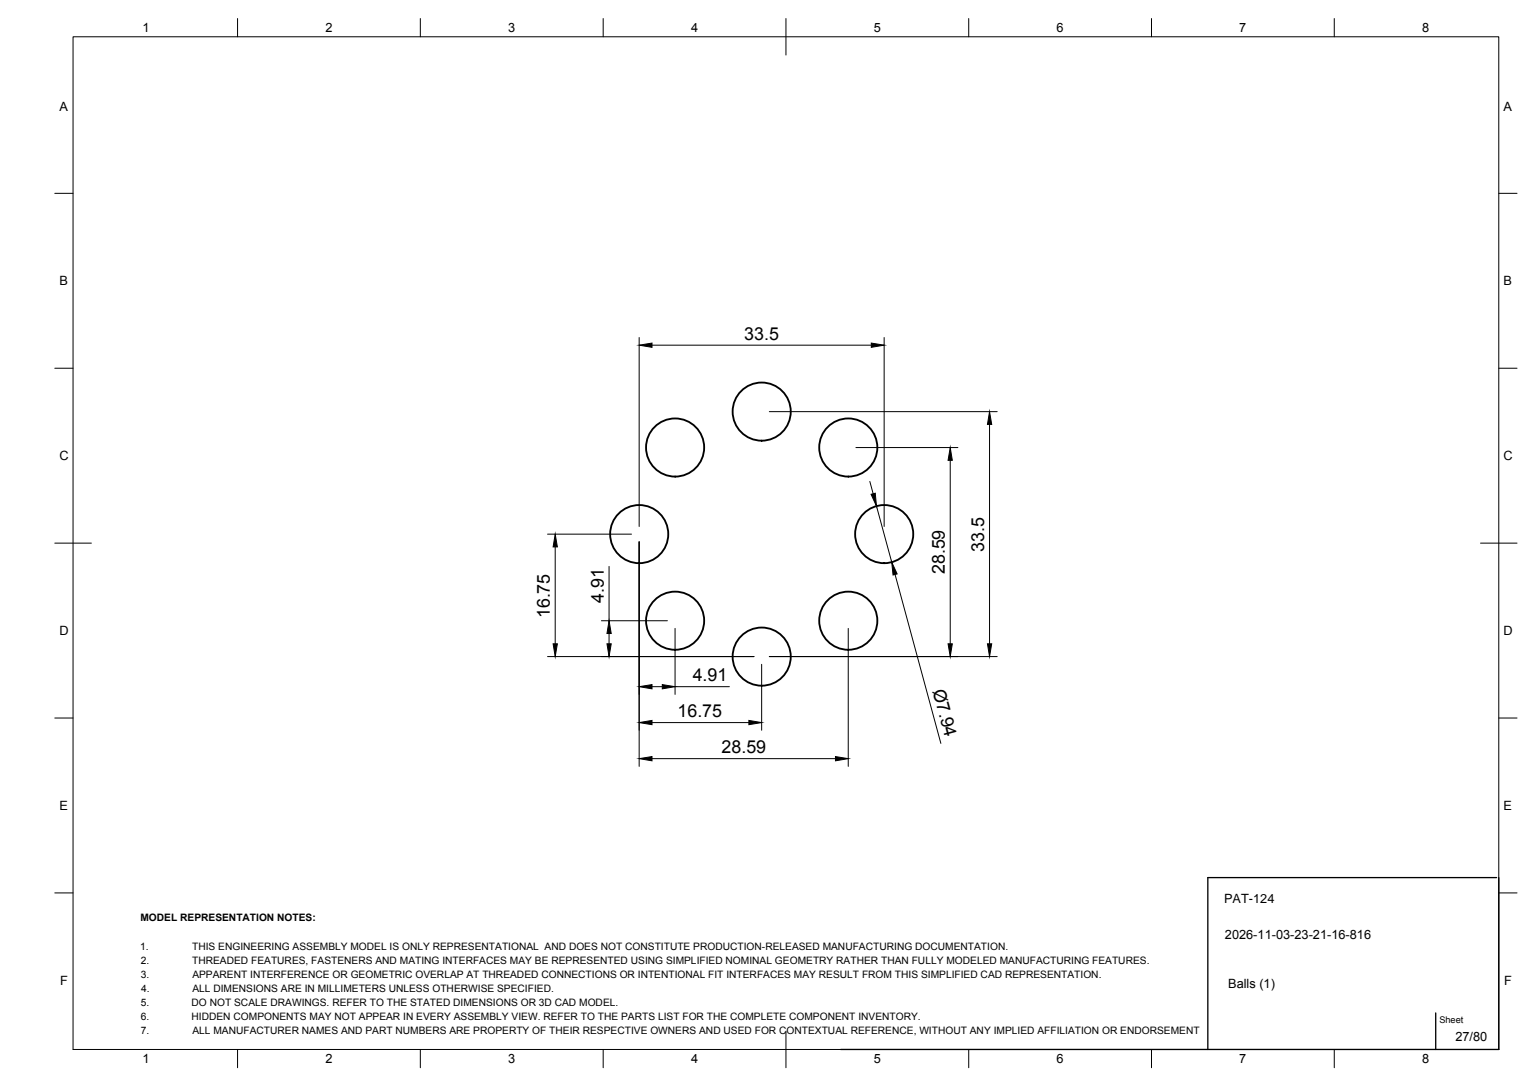
ISO-10303-21;
HEADER;
/* Generated by software containing ST-Developer
 * from STEP Tools, Inc. (www.steptools.com) 
 */

FILE_DESCRIPTION(
/* description */ ('XY cross-slide table'),
/* implementation_level */ '2;1');

FILE_NAME(
/* name */ 'Balls (1).step',
/* time_stamp */ '2026-10-28T03:22:46-07:00',
/* author */ (''),
/* organization */ (''),
/* preprocessor_version */ 'ST-DEVELOPER v20.2',
/* originating_system */ 'Autodesk Translation Framework v15.17.0.0',
/* authorisation */ '');

FILE_SCHEMA (('AUTOMOTIVE_DESIGN { 1 0 10303 214 3 1 1 }'));
ENDSEC;

DATA;
#10=MECHANICAL_DESIGN_GEOMETRIC_PRESENTATION_REPRESENTATION('',(#1695,#1696,#1697,#1698,#1699,#1700,#1701,#1702),#62984);
#1395=SPHERICAL_SURFACE('',#24455,0.3969);
#1396=SPHERICAL_SURFACE('',#24457,0.3969);
#1397=SPHERICAL_SURFACE('',#24459,0.3969);
#1398=SPHERICAL_SURFACE('',#24461,0.3969);
#1399=SPHERICAL_SURFACE('',#24463,0.3969);
#1400=SPHERICAL_SURFACE('',#24465,0.3969);
#1401=SPHERICAL_SURFACE('',#24467,0.3969);
#1402=SPHERICAL_SURFACE('',#24469,0.3969);
#1522=SHAPE_REPRESENTATION_RELATIONSHIP('SRR','None',#63372,#1605);
#1605=ADVANCED_BREP_SHAPE_REPRESENTATION('',(#1808,#1809,#1810,#1811,#1812,
#1813,#1814,#1815),#62909);
#1695=STYLED_ITEM('',(#63912),#1808);
#1696=STYLED_ITEM('',(#63912),#1809);
#1697=STYLED_ITEM('',(#63912),#1810);
#1698=STYLED_ITEM('',(#63912),#1811);
#1699=STYLED_ITEM('',(#63912),#1812);
#1700=STYLED_ITEM('',(#63912),#1813);
#1701=STYLED_ITEM('',(#63912),#1814);
#1702=STYLED_ITEM('',(#63912),#1815);
#1808=MANIFOLD_SOLID_BREP('Body1',#22989);
#1809=MANIFOLD_SOLID_BREP('Body2',#22990);
#1810=MANIFOLD_SOLID_BREP('Body3',#22991);
#1811=MANIFOLD_SOLID_BREP('Body4',#22992);
#1812=MANIFOLD_SOLID_BREP('Body5',#22993);
#1813=MANIFOLD_SOLID_BREP('Body6',#22994);
#1814=MANIFOLD_SOLID_BREP('Body7',#22995);
#1815=MANIFOLD_SOLID_BREP('Body8',#22996);
#3080=FACE_OUTER_BOUND('',#4503,.T.);
#3081=FACE_OUTER_BOUND('',#4504,.T.);
#3082=FACE_OUTER_BOUND('',#4505,.T.);
#3083=FACE_OUTER_BOUND('',#4506,.T.);
#3084=FACE_OUTER_BOUND('',#4507,.T.);
#3085=FACE_OUTER_BOUND('',#4508,.T.);
#3086=FACE_OUTER_BOUND('',#4509,.T.);
#3087=FACE_OUTER_BOUND('',#4510,.T.);
#4503=EDGE_LOOP('',(#15816,#15817));
#4504=EDGE_LOOP('',(#15818,#15819));
#4505=EDGE_LOOP('',(#15820,#15821));
#4506=EDGE_LOOP('',(#15822,#15823));
#4507=EDGE_LOOP('',(#15824,#15825));
#4508=EDGE_LOOP('',(#15826,#15827));
#4509=EDGE_LOOP('',(#15828,#15829));
#4510=EDGE_LOOP('',(#15830,#15831));
#9095=CIRCLE('',#24456,0.3969);
#9096=CIRCLE('',#24458,0.3969);
#9097=CIRCLE('',#24460,0.3969);
#9098=CIRCLE('',#24462,0.3969);
#9099=CIRCLE('',#24464,0.3969);
#9100=CIRCLE('',#24466,0.3969);
#9101=CIRCLE('',#24468,0.3969);
#9102=CIRCLE('',#24470,0.3969);
#10081=VERTEX_POINT('',#34169);
#10082=VERTEX_POINT('',#34170);
#10083=VERTEX_POINT('',#34173);
#10084=VERTEX_POINT('',#34174);
#10085=VERTEX_POINT('',#34177);
#10086=VERTEX_POINT('',#34178);
#10087=VERTEX_POINT('',#34181);
#10088=VERTEX_POINT('',#34182);
#10089=VERTEX_POINT('',#34185);
#10090=VERTEX_POINT('',#34186);
#10091=VERTEX_POINT('',#34189);
#10092=VERTEX_POINT('',#34190);
#10093=VERTEX_POINT('',#34193);
#10094=VERTEX_POINT('',#34194);
#10095=VERTEX_POINT('',#34197);
#10096=VERTEX_POINT('',#34198);
#12292=EDGE_CURVE('',#10081,#10082,#9095,.T.);
#12293=EDGE_CURVE('',#10083,#10084,#9096,.T.);
#12294=EDGE_CURVE('',#10085,#10086,#9097,.T.);
#12295=EDGE_CURVE('',#10087,#10088,#9098,.T.);
#12296=EDGE_CURVE('',#10089,#10090,#9099,.T.);
#12297=EDGE_CURVE('',#10091,#10092,#9100,.T.);
#12298=EDGE_CURVE('',#10093,#10094,#9101,.T.);
#12299=EDGE_CURVE('',#10095,#10096,#9102,.T.);
#15816=ORIENTED_EDGE('',*,*,#12292,.T.);
#15817=ORIENTED_EDGE('',*,*,#12292,.F.);
#15818=ORIENTED_EDGE('',*,*,#12293,.T.);
#15819=ORIENTED_EDGE('',*,*,#12293,.F.);
#15820=ORIENTED_EDGE('',*,*,#12294,.T.);
#15821=ORIENTED_EDGE('',*,*,#12294,.F.);
#15822=ORIENTED_EDGE('',*,*,#12295,.T.);
#15823=ORIENTED_EDGE('',*,*,#12295,.F.);
#15824=ORIENTED_EDGE('',*,*,#12296,.T.);
#15825=ORIENTED_EDGE('',*,*,#12296,.F.);
#15826=ORIENTED_EDGE('',*,*,#12297,.T.);
#15827=ORIENTED_EDGE('',*,*,#12297,.F.);
#15828=ORIENTED_EDGE('',*,*,#12298,.T.);
#15829=ORIENTED_EDGE('',*,*,#12298,.F.);
#15830=ORIENTED_EDGE('',*,*,#12299,.T.);
#15831=ORIENTED_EDGE('',*,*,#12299,.F.);
#21861=ADVANCED_FACE('',(#3080),#1395,.T.);
#21862=ADVANCED_FACE('',(#3081),#1396,.T.);
#21863=ADVANCED_FACE('',(#3082),#1397,.T.);
#21864=ADVANCED_FACE('',(#3083),#1398,.T.);
#21865=ADVANCED_FACE('',(#3084),#1399,.T.);
#21866=ADVANCED_FACE('',(#3085),#1400,.T.);
#21867=ADVANCED_FACE('',(#3086),#1401,.T.);
#21868=ADVANCED_FACE('',(#3087),#1402,.T.);
#22989=CLOSED_SHELL('',(#21861));
#22990=CLOSED_SHELL('',(#21862));
#22991=CLOSED_SHELL('',(#21863));
#22992=CLOSED_SHELL('',(#21864));
#22993=CLOSED_SHELL('',(#21865));
#22994=CLOSED_SHELL('',(#21866));
#22995=CLOSED_SHELL('',(#21867));
#22996=CLOSED_SHELL('',(#21868));
#24454=AXIS2_PLACEMENT_3D('',#34167,#27596,#27597);
#24455=AXIS2_PLACEMENT_3D('',#34168,#27598,#27599);
#24456=AXIS2_PLACEMENT_3D('',#34171,#27600,#27601);
#24457=AXIS2_PLACEMENT_3D('',#34172,#27602,#27603);
#24458=AXIS2_PLACEMENT_3D('',#34175,#27604,#27605);
#24459=AXIS2_PLACEMENT_3D('',#34176,#27606,#27607);
#24460=AXIS2_PLACEMENT_3D('',#34179,#27608,#27609);
#24461=AXIS2_PLACEMENT_3D('',#34180,#27610,#27611);
#24462=AXIS2_PLACEMENT_3D('',#34183,#27612,#27613);
#24463=AXIS2_PLACEMENT_3D('',#34184,#27614,#27615);
#24464=AXIS2_PLACEMENT_3D('',#34187,#27616,#27617);
#24465=AXIS2_PLACEMENT_3D('',#34188,#27618,#27619);
#24466=AXIS2_PLACEMENT_3D('',#34191,#27620,#27621);
#24467=AXIS2_PLACEMENT_3D('',#34192,#27622,#27623);
#24468=AXIS2_PLACEMENT_3D('',#34195,#27624,#27625);
#24469=AXIS2_PLACEMENT_3D('',#34196,#27626,#27627);
#24470=AXIS2_PLACEMENT_3D('',#34199,#27628,#27629);
#27596=DIRECTION('axis',(0.,0.,1.));
#27597=DIRECTION('refdir',(1.,0.,0.));
#27598=DIRECTION('center_axis',(0.,0.,1.));
#27599=DIRECTION('ref_axis',(1.,0.,0.));
#27600=DIRECTION('center_axis',(1.22464679914735E-16,-1.,0.));
#27601=DIRECTION('ref_axis',(-1.,-1.22464679914735E-16,0.));
#27602=DIRECTION('center_axis',(0.707106781186548,0.,0.707106781186548));
#27603=DIRECTION('ref_axis',(0.707106781186548,0.,-0.707106781186548));
#27604=DIRECTION('center_axis',(8.65956056235493E-17,-1.,-8.65956056235493E-17));
#27605=DIRECTION('ref_axis',(-0.707106781186548,-1.22464679914735E-16,0.707106781186548));
#27606=DIRECTION('center_axis',(1.,0.,0.));
#27607=DIRECTION('ref_axis',(6.12323399573677E-17,0.,-1.));
#27608=DIRECTION('center_axis',(7.49879891330929E-33,-1.,-1.22464679914735E-16));
#27609=DIRECTION('ref_axis',(-6.12323399573677E-17,-1.22464679914735E-16,
1.));
#27610=DIRECTION('center_axis',(0.707106781186548,0.,-0.707106781186548));
#27611=DIRECTION('ref_axis',(-0.707106781186548,0.,-0.707106781186548));
#27612=DIRECTION('center_axis',(-8.65956056235493E-17,-1.,-8.65956056235493E-17));
#27613=DIRECTION('ref_axis',(0.707106781186548,-1.22464679914735E-16,0.707106781186548));
#27614=DIRECTION('center_axis',(0.,0.,-1.));
#27615=DIRECTION('ref_axis',(-1.,0.,-1.22464679914735E-16));
#27616=DIRECTION('center_axis',(-1.22464679914735E-16,-1.,-1.49975978266186E-32));
#27617=DIRECTION('ref_axis',(1.,-1.22464679914735E-16,1.22464679914735E-16));
#27618=DIRECTION('center_axis',(-0.707106781186548,0.,-0.707106781186548));
#27619=DIRECTION('ref_axis',(-0.707106781186548,0.,0.707106781186548));
#27620=DIRECTION('center_axis',(-8.65956056235493E-17,-1.,8.65956056235493E-17));
#27621=DIRECTION('ref_axis',(0.707106781186548,-1.22464679914735E-16,-0.707106781186548));
#27622=DIRECTION('center_axis',(-1.,0.,0.));
#27623=DIRECTION('ref_axis',(-1.83697019872103E-16,0.,1.));
#27624=DIRECTION('center_axis',(-2.24963967399279E-32,-1.,1.22464679914735E-16));
#27625=DIRECTION('ref_axis',(1.83697019872103E-16,-1.22464679914735E-16,
-1.));
#27626=DIRECTION('center_axis',(-0.707106781186548,0.,0.707106781186548));
#27627=DIRECTION('ref_axis',(0.707106781186548,0.,0.707106781186548));
#27628=DIRECTION('center_axis',(8.65956056235493E-17,-1.,8.65956056235494E-17));
#27629=DIRECTION('ref_axis',(-0.707106781186548,-1.22464679914735E-16,-0.707106781186548));
#34167=CARTESIAN_POINT('',(0.,0.,0.));
#34168=CARTESIAN_POINT('Origin',(1.675,0.,0.));
#34169=CARTESIAN_POINT('',(1.675,-2.97627328869245E-33,0.3969));
#34170=CARTESIAN_POINT('',(1.675,-2.97627328869245E-33,-0.3969));
#34171=CARTESIAN_POINT('Origin',(1.675,0.,0.));
#34172=CARTESIAN_POINT('Origin',(1.18440385848747,0.,-1.18440385848747));
#34173=CARTESIAN_POINT('',(1.46505453994041,3.1867025333467E-33,-0.903753177034526));
#34174=CARTESIAN_POINT('',(0.903753177034527,-9.13924911073161E-33,-1.46505453994041));
#34175=CARTESIAN_POINT('Origin',(1.18440385848747,0.,-1.18440385848747));
#34176=CARTESIAN_POINT('Origin',(1.02564169428591E-16,0.,-1.675));
#34177=CARTESIAN_POINT('',(0.3969,-2.97627328869246E-33,-1.675));
#34178=CARTESIAN_POINT('',(-0.3969,-2.97627328869245E-33,-1.675));
#34179=CARTESIAN_POINT('Origin',(1.02564169428591E-16,0.,-1.675));
#34180=CARTESIAN_POINT('Origin',(-1.18440385848747,0.,-1.18440385848747));
#34181=CARTESIAN_POINT('',(-0.903753177034526,3.1867025333467E-33,-1.46505453994041));
#34182=CARTESIAN_POINT('',(-1.46505453994041,-9.13924911073161E-33,-0.903753177034527));
#34183=CARTESIAN_POINT('Origin',(-1.18440385848747,0.,-1.18440385848747));
#34184=CARTESIAN_POINT('Origin',(-1.675,0.,-2.05128338857182E-16));
#34185=CARTESIAN_POINT('',(-1.675,-2.97627328869246E-33,-0.3969));
#34186=CARTESIAN_POINT('',(-1.675,-2.97627328869245E-33,0.3969));
#34187=CARTESIAN_POINT('Origin',(-1.675,0.,-2.05128338857182E-16));
#34188=CARTESIAN_POINT('Origin',(-1.18440385848747,0.,1.18440385848747));
#34189=CARTESIAN_POINT('',(-1.46505453994041,6.26819044436628E-33,0.903753177034526));
#34190=CARTESIAN_POINT('',(-0.903753177034527,-1.22207370217512E-32,1.46505453994041));
#34191=CARTESIAN_POINT('Origin',(-1.18440385848747,0.,1.18440385848747));
#34192=CARTESIAN_POINT('Origin',(-3.07692508285772E-16,0.,1.675));
#34193=CARTESIAN_POINT('',(-0.3969,-2.97627328869246E-33,1.675));
#34194=CARTESIAN_POINT('',(0.396899999999999,-2.97627328869245E-33,1.675));
#34195=CARTESIAN_POINT('Origin',(-3.07692508285772E-16,0.,1.675));
#34196=CARTESIAN_POINT('Origin',(1.18440385848747,0.,1.18440385848747));
#34197=CARTESIAN_POINT('',(0.903753177034526,9.34967835538585E-33,1.46505453994041));
#34198=CARTESIAN_POINT('',(1.46505453994041,-1.53022249327708E-32,0.903753177034527));
#34199=CARTESIAN_POINT('Origin',(1.18440385848747,0.,1.18440385848747));
#62810=UNCERTAINTY_MEASURE_WITH_UNIT(LENGTH_MEASURE(0.001),#62985,
'DISTANCE_ACCURACY_VALUE',
'Maximum model space distance between geometric entities at asserted c
onnectivities');
#62885=UNCERTAINTY_MEASURE_WITH_UNIT(LENGTH_MEASURE(0.001),#62985,
'DISTANCE_ACCURACY_VALUE',
'Maximum model space distance between geometric entities at asserted c
onnectivities');
#62909=(
GEOMETRIC_REPRESENTATION_CONTEXT(3)
GLOBAL_UNCERTAINTY_ASSIGNED_CONTEXT((#62810))
GLOBAL_UNIT_ASSIGNED_CONTEXT((#62985,#62987,#62988))
REPRESENTATION_CONTEXT('','3D')
);
#62984=(
GEOMETRIC_REPRESENTATION_CONTEXT(3)
GLOBAL_UNCERTAINTY_ASSIGNED_CONTEXT((#62885))
GLOBAL_UNIT_ASSIGNED_CONTEXT((#62985,#62987,#62988))
REPRESENTATION_CONTEXT('','3D')
);
#62985=(
LENGTH_UNIT()
NAMED_UNIT(*)
SI_UNIT(.CENTI.,.METRE.)
);
#62987=(
NAMED_UNIT(*)
PLANE_ANGLE_UNIT()
SI_UNIT($,.RADIAN.)
);
#62988=(
NAMED_UNIT(*)
SI_UNIT($,.STERADIAN.)
SOLID_ANGLE_UNIT()
);
#63012=SHAPE_DEFINITION_REPRESENTATION(#63115,#63372);
#63115=PRODUCT_DEFINITION_SHAPE('',$,#63471);
#63372=SHAPE_REPRESENTATION('',(#24454),#62909);
#63447=PRODUCT_DEFINITION_CONTEXT('part definition',#63743,'design');
#63471=PRODUCT_DEFINITION('Balls (1)','Balls (1)',#63569,#63447);
#63569=PRODUCT_DEFINITION_FORMATION('',$,#63768);
#63743=APPLICATION_CONTEXT(
'Core Data for Automotive Mechanical Design Process');
#63744=PRODUCT_CONTEXT('part definition',#63743,'mechanical');
#63768=PRODUCT('Balls (1)','Balls (1)','Balls (1)',(#63744));
#63906=COLOUR_RGB('Grey',0.48,0.52,0.57);
#63907=FILL_AREA_STYLE_COLOUR('',#63906);
#63908=FILL_AREA_STYLE('',(#63907));
#63909=SURFACE_STYLE_FILL_AREA(#63908);
#63910=SURFACE_SIDE_STYLE('',(#63909));
#63911=SURFACE_STYLE_USAGE(.BOTH.,#63910);
#63912=PRESENTATION_STYLE_ASSIGNMENT((#63911));
ENDSEC;
END-ISO-10303-21;
